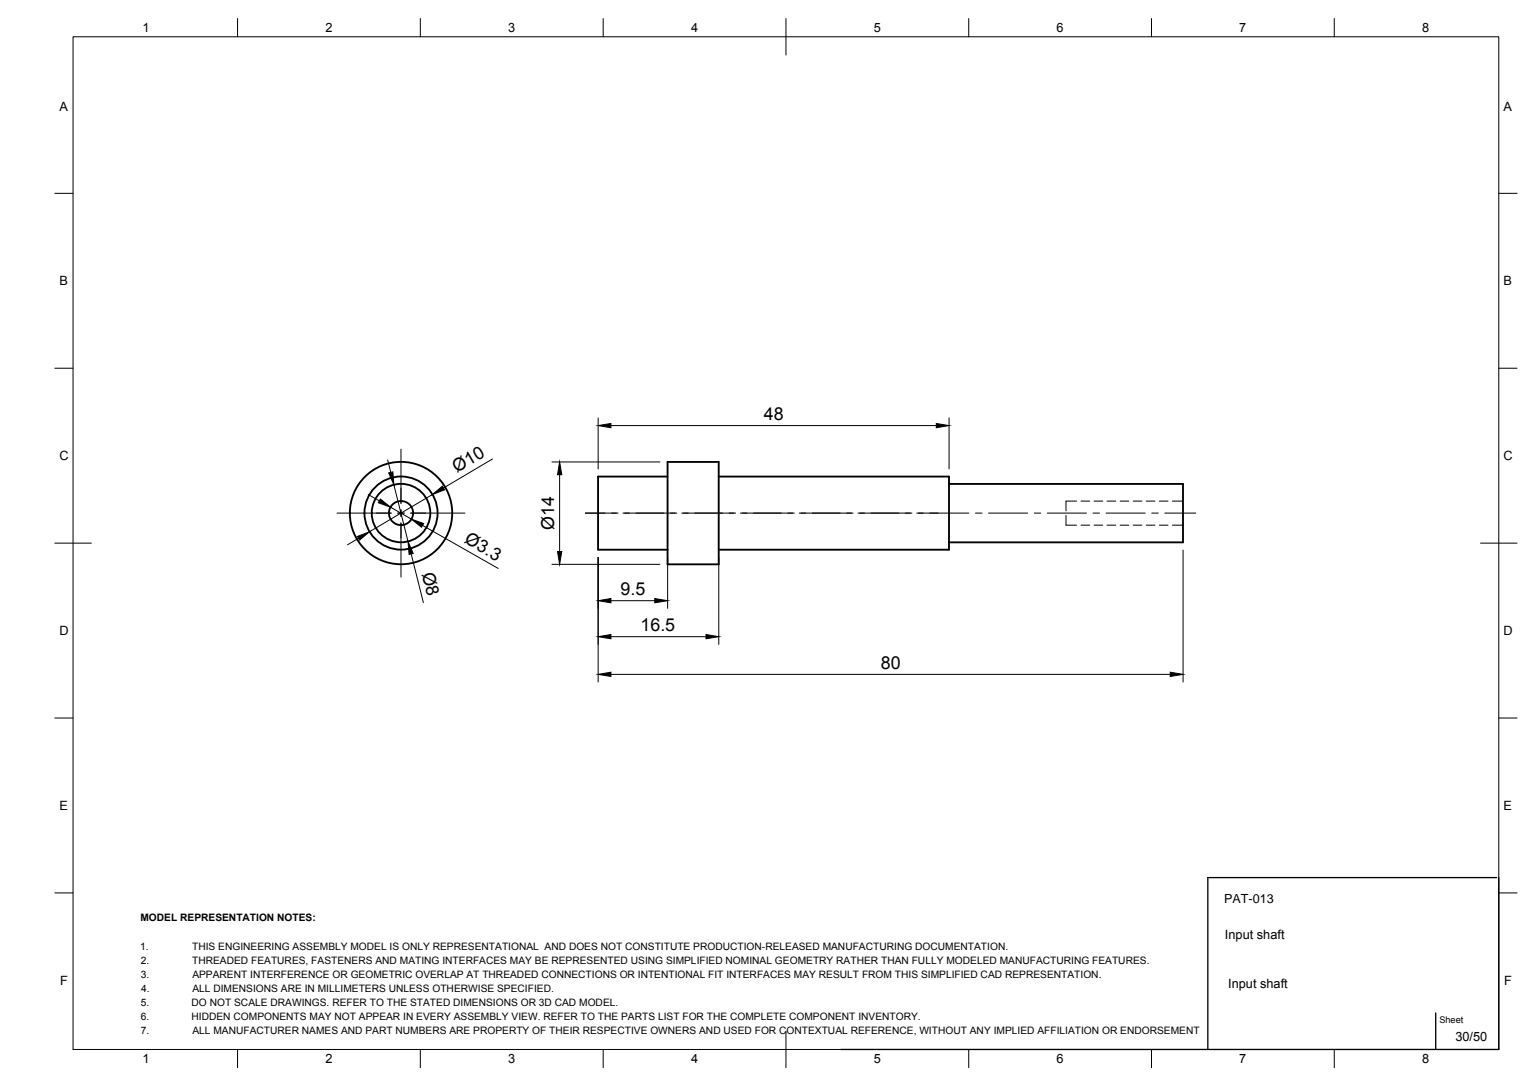
ISO-10303-21;
HEADER;
/* Generated by software containing ST-Developer
 * from STEP Tools, Inc. (www.steptools.com) 
 */

FILE_DESCRIPTION(
/* description */ ('Belt-driven linear axis on 2020 extrusion'),
/* implementation_level */ '2;1');

FILE_NAME(
/* name */ 'Input shaft.step',
/* time_stamp */ '2026-10-28T03:26:09-07:00',
/* author */ (''),
/* organization */ (''),
/* preprocessor_version */ 'ST-DEVELOPER v20.2',
/* originating_system */ 'Autodesk Translation Framework v15.17.0.0',
/* authorisation */ '');

FILE_SCHEMA (('AUTOMOTIVE_DESIGN { 1 0 10303 214 3 1 1 }'));
ENDSEC;

DATA;
#10=MECHANICAL_DESIGN_GEOMETRIC_PRESENTATION_REPRESENTATION('',(#643),#20096);
#541=SHAPE_REPRESENTATION_RELATIONSHIP('SRR','None',#20339,#587);
#587=ADVANCED_BREP_SHAPE_REPRESENTATION('',(#698),#20070);
#643=STYLED_ITEM('',(#20650),#698);
#698=MANIFOLD_SOLID_BREP('Body1',#10957);
#829=FACE_BOUND('',#2354,.T.);
#830=FACE_BOUND('',#2356,.T.);
#831=FACE_BOUND('',#2361,.T.);
#832=FACE_BOUND('',#2365,.T.);
#1110=PLANE('',#12193);
#1111=PLANE('',#12194);
#1112=PLANE('',#12197);
#1113=PLANE('',#12206);
#1114=PLANE('',#12209);
#1115=PLANE('',#12210);
#1618=FACE_OUTER_BOUND('',#2351,.T.);
#1619=FACE_OUTER_BOUND('',#2352,.T.);
#1620=FACE_OUTER_BOUND('',#2353,.T.);
#1621=FACE_OUTER_BOUND('',#2355,.T.);
#1622=FACE_OUTER_BOUND('',#2357,.T.);
#1623=FACE_OUTER_BOUND('',#2358,.T.);
#1624=FACE_OUTER_BOUND('',#2359,.T.);
#1625=FACE_OUTER_BOUND('',#2360,.T.);
#1626=FACE_OUTER_BOUND('',#2362,.T.);
#1627=FACE_OUTER_BOUND('',#2363,.T.);
#1628=FACE_OUTER_BOUND('',#2364,.T.);
#2351=EDGE_LOOP('',(#8965,#8966,#8967,#8968));
#2352=EDGE_LOOP('',(#8969));
#2353=EDGE_LOOP('',(#8970));
#2354=EDGE_LOOP('',(#8971));
#2355=EDGE_LOOP('',(#8972));
#2356=EDGE_LOOP('',(#8973));
#2357=EDGE_LOOP('',(#8974,#8975,#8976,#8977));
#2358=EDGE_LOOP('',(#8978,#8979,#8980,#8981));
#2359=EDGE_LOOP('',(#8982,#8983,#8984,#8985));
#2360=EDGE_LOOP('',(#8986));
#2361=EDGE_LOOP('',(#8987));
#2362=EDGE_LOOP('',(#8988,#8989,#8990,#8991));
#2363=EDGE_LOOP('',(#8992));
#2364=EDGE_LOOP('',(#8993));
#2365=EDGE_LOOP('',(#8994));
#3204=LINE('',#18410,#4061);
#3205=LINE('',#18424,#4062);
#3206=LINE('',#18427,#4063);
#3207=LINE('',#18433,#4064);
#3208=LINE('',#18439,#4065);
#4061=VECTOR('',#14728,0.165);
#4062=VECTOR('',#14747,0.7);
#4063=VECTOR('',#14750,0.5);
#4064=VECTOR('',#14757,0.4);
#4065=VECTOR('',#14766,0.5);
#4676=CIRCLE('',#12191,0.165);
#4677=CIRCLE('',#12192,0.165);
#4678=CIRCLE('',#12195,0.7);
#4679=CIRCLE('',#12196,0.5);
#4680=CIRCLE('',#12198,0.7);
#4681=CIRCLE('',#12199,0.5);
#4682=CIRCLE('',#12202,0.5);
#4683=CIRCLE('',#12204,0.4);
#4684=CIRCLE('',#12205,0.4);
#4685=CIRCLE('',#12208,0.5);
#5471=VERTEX_POINT('',#18407);
#5472=VERTEX_POINT('',#18409);
#5473=VERTEX_POINT('',#18414);
#5474=VERTEX_POINT('',#18416);
#5475=VERTEX_POINT('',#18419);
#5476=VERTEX_POINT('',#18421);
#5477=VERTEX_POINT('',#18426);
#5478=VERTEX_POINT('',#18430);
#5479=VERTEX_POINT('',#18432);
#5480=VERTEX_POINT('',#18437);
#6697=EDGE_CURVE('',#5471,#5471,#4676,.T.);
#6698=EDGE_CURVE('',#5471,#5472,#3204,.T.);
#6699=EDGE_CURVE('',#5472,#5472,#4677,.T.);
#6700=EDGE_CURVE('',#5473,#5473,#4678,.T.);
#6701=EDGE_CURVE('',#5474,#5474,#4679,.T.);
#6702=EDGE_CURVE('',#5475,#5475,#4680,.T.);
#6703=EDGE_CURVE('',#5476,#5476,#4681,.T.);
#6704=EDGE_CURVE('',#5473,#5475,#3205,.T.);
#6705=EDGE_CURVE('',#5476,#5477,#3206,.T.);
#6706=EDGE_CURVE('',#5477,#5477,#4682,.T.);
#6707=EDGE_CURVE('',#5478,#5478,#4683,.T.);
#6708=EDGE_CURVE('',#5478,#5479,#3207,.T.);
#6709=EDGE_CURVE('',#5479,#5479,#4684,.T.);
#6710=EDGE_CURVE('',#5480,#5480,#4685,.T.);
#6711=EDGE_CURVE('',#5480,#5474,#3208,.T.);
#8965=ORIENTED_EDGE('',*,*,#6697,.F.);
#8966=ORIENTED_EDGE('',*,*,#6698,.T.);
#8967=ORIENTED_EDGE('',*,*,#6699,.T.);
#8968=ORIENTED_EDGE('',*,*,#6698,.F.);
#8969=ORIENTED_EDGE('',*,*,#6699,.F.);
#8970=ORIENTED_EDGE('',*,*,#6700,.T.);
#8971=ORIENTED_EDGE('',*,*,#6701,.F.);
#8972=ORIENTED_EDGE('',*,*,#6702,.F.);
#8973=ORIENTED_EDGE('',*,*,#6703,.F.);
#8974=ORIENTED_EDGE('',*,*,#6700,.F.);
#8975=ORIENTED_EDGE('',*,*,#6704,.T.);
#8976=ORIENTED_EDGE('',*,*,#6702,.T.);
#8977=ORIENTED_EDGE('',*,*,#6704,.F.);
#8978=ORIENTED_EDGE('',*,*,#6703,.T.);
#8979=ORIENTED_EDGE('',*,*,#6705,.T.);
#8980=ORIENTED_EDGE('',*,*,#6706,.T.);
#8981=ORIENTED_EDGE('',*,*,#6705,.F.);
#8982=ORIENTED_EDGE('',*,*,#6707,.F.);
#8983=ORIENTED_EDGE('',*,*,#6708,.T.);
#8984=ORIENTED_EDGE('',*,*,#6709,.T.);
#8985=ORIENTED_EDGE('',*,*,#6708,.F.);
#8986=ORIENTED_EDGE('',*,*,#6709,.F.);
#8987=ORIENTED_EDGE('',*,*,#6697,.T.);
#8988=ORIENTED_EDGE('',*,*,#6710,.F.);
#8989=ORIENTED_EDGE('',*,*,#6711,.T.);
#8990=ORIENTED_EDGE('',*,*,#6701,.T.);
#8991=ORIENTED_EDGE('',*,*,#6711,.F.);
#8992=ORIENTED_EDGE('',*,*,#6710,.T.);
#8993=ORIENTED_EDGE('',*,*,#6706,.F.);
#8994=ORIENTED_EDGE('',*,*,#6707,.T.);
#10199=CYLINDRICAL_SURFACE('',#12190,0.165);
#10200=CYLINDRICAL_SURFACE('',#12200,0.7);
#10201=CYLINDRICAL_SURFACE('',#12201,0.5);
#10202=CYLINDRICAL_SURFACE('',#12203,0.4);
#10203=CYLINDRICAL_SURFACE('',#12207,0.5);
#10669=ADVANCED_FACE('',(#1618),#10199,.F.);
#10670=ADVANCED_FACE('',(#1619),#1110,.F.);
#10671=ADVANCED_FACE('',(#1620,#829),#1111,.T.);
#10672=ADVANCED_FACE('',(#1621,#830),#1112,.F.);
#10673=ADVANCED_FACE('',(#1622),#10200,.T.);
#10674=ADVANCED_FACE('',(#1623),#10201,.T.);
#10675=ADVANCED_FACE('',(#1624),#10202,.T.);
#10676=ADVANCED_FACE('',(#1625,#831),#1113,.F.);
#10677=ADVANCED_FACE('',(#1626),#10203,.T.);
#10678=ADVANCED_FACE('',(#1627),#1114,.T.);
#10679=ADVANCED_FACE('',(#1628,#832),#1115,.F.);
#10957=CLOSED_SHELL('',(#10669,#10670,#10671,#10672,#10673,#10674,#10675,
#10676,#10677,#10678,#10679));
#12189=AXIS2_PLACEMENT_3D('',#18405,#14722,#14723);
#12190=AXIS2_PLACEMENT_3D('',#18406,#14724,#14725);
#12191=AXIS2_PLACEMENT_3D('',#18408,#14726,#14727);
#12192=AXIS2_PLACEMENT_3D('',#18411,#14729,#14730);
#12193=AXIS2_PLACEMENT_3D('',#18412,#14731,#14732);
#12194=AXIS2_PLACEMENT_3D('',#18413,#14733,#14734);
#12195=AXIS2_PLACEMENT_3D('',#18415,#14735,#14736);
#12196=AXIS2_PLACEMENT_3D('',#18417,#14737,#14738);
#12197=AXIS2_PLACEMENT_3D('',#18418,#14739,#14740);
#12198=AXIS2_PLACEMENT_3D('',#18420,#14741,#14742);
#12199=AXIS2_PLACEMENT_3D('',#18422,#14743,#14744);
#12200=AXIS2_PLACEMENT_3D('',#18423,#14745,#14746);
#12201=AXIS2_PLACEMENT_3D('',#18425,#14748,#14749);
#12202=AXIS2_PLACEMENT_3D('',#18428,#14751,#14752);
#12203=AXIS2_PLACEMENT_3D('',#18429,#14753,#14754);
#12204=AXIS2_PLACEMENT_3D('',#18431,#14755,#14756);
#12205=AXIS2_PLACEMENT_3D('',#18434,#14758,#14759);
#12206=AXIS2_PLACEMENT_3D('',#18435,#14760,#14761);
#12207=AXIS2_PLACEMENT_3D('',#18436,#14762,#14763);
#12208=AXIS2_PLACEMENT_3D('',#18438,#14764,#14765);
#12209=AXIS2_PLACEMENT_3D('',#18440,#14767,#14768);
#12210=AXIS2_PLACEMENT_3D('',#18441,#14769,#14770);
#14722=DIRECTION('axis',(0.,0.,1.));
#14723=DIRECTION('refdir',(1.,0.,0.));
#14724=DIRECTION('center_axis',(0.,1.,0.));
#14725=DIRECTION('ref_axis',(1.,0.,0.));
#14726=DIRECTION('center_axis',(0.,1.,0.));
#14727=DIRECTION('ref_axis',(1.,0.,0.));
#14728=DIRECTION('',(0.,1.,0.));
#14729=DIRECTION('center_axis',(0.,1.,0.));
#14730=DIRECTION('ref_axis',(1.,0.,0.));
#14731=DIRECTION('center_axis',(0.,1.,0.));
#14732=DIRECTION('ref_axis',(1.,0.,0.));
#14733=DIRECTION('center_axis',(0.,1.,0.));
#14734=DIRECTION('ref_axis',(1.,0.,0.));
#14735=DIRECTION('center_axis',(0.,1.,0.));
#14736=DIRECTION('ref_axis',(1.,0.,0.));
#14737=DIRECTION('center_axis',(0.,1.,0.));
#14738=DIRECTION('ref_axis',(1.,0.,0.));
#14739=DIRECTION('center_axis',(0.,1.,0.));
#14740=DIRECTION('ref_axis',(1.,0.,0.));
#14741=DIRECTION('center_axis',(0.,1.,0.));
#14742=DIRECTION('ref_axis',(1.,0.,0.));
#14743=DIRECTION('center_axis',(0.,-1.,0.));
#14744=DIRECTION('ref_axis',(1.,0.,0.));
#14745=DIRECTION('center_axis',(0.,1.,0.));
#14746=DIRECTION('ref_axis',(1.,0.,0.));
#14747=DIRECTION('',(0.,-1.,0.));
#14748=DIRECTION('center_axis',(0.,1.,0.));
#14749=DIRECTION('ref_axis',(1.,0.,0.));
#14750=DIRECTION('',(0.,-1.,0.));
#14751=DIRECTION('center_axis',(0.,1.,0.));
#14752=DIRECTION('ref_axis',(1.,0.,0.));
#14753=DIRECTION('center_axis',(0.,1.,0.));
#14754=DIRECTION('ref_axis',(1.,0.,0.));
#14755=DIRECTION('center_axis',(0.,1.,0.));
#14756=DIRECTION('ref_axis',(1.,0.,0.));
#14757=DIRECTION('',(0.,-1.,0.));
#14758=DIRECTION('center_axis',(0.,1.,0.));
#14759=DIRECTION('ref_axis',(1.,0.,0.));
#14760=DIRECTION('center_axis',(0.,1.,0.));
#14761=DIRECTION('ref_axis',(1.,0.,0.));
#14762=DIRECTION('center_axis',(0.,1.,0.));
#14763=DIRECTION('ref_axis',(1.,0.,0.));
#14764=DIRECTION('center_axis',(0.,1.,0.));
#14765=DIRECTION('ref_axis',(1.,0.,0.));
#14766=DIRECTION('',(0.,-1.,0.));
#14767=DIRECTION('center_axis',(0.,1.,0.));
#14768=DIRECTION('ref_axis',(1.,0.,0.));
#14769=DIRECTION('center_axis',(0.,1.,0.));
#14770=DIRECTION('ref_axis',(1.,0.,0.));
#18405=CARTESIAN_POINT('',(0.,0.,0.));
#18406=CARTESIAN_POINT('Origin',(0.,-5.1,7.));
#18407=CARTESIAN_POINT('',(-0.165,-5.,7.));
#18408=CARTESIAN_POINT('Origin',(0.,-5.,7.));
#18409=CARTESIAN_POINT('',(-0.165,-3.4,7.));
#18410=CARTESIAN_POINT('',(-0.165,-5.1,7.));
#18411=CARTESIAN_POINT('Origin',(0.,-3.4,7.));
#18412=CARTESIAN_POINT('Origin',(0.,-3.4,7.));
#18413=CARTESIAN_POINT('Origin',(0.,2.05,7.));
#18414=CARTESIAN_POINT('',(-0.7,2.05,7.));
#18415=CARTESIAN_POINT('Origin',(0.,2.05,7.));
#18416=CARTESIAN_POINT('',(-0.5,2.05,7.));
#18417=CARTESIAN_POINT('Origin',(0.,2.05,7.));
#18418=CARTESIAN_POINT('Origin',(0.,1.35,7.));
#18419=CARTESIAN_POINT('',(-0.7,1.35,7.));
#18420=CARTESIAN_POINT('Origin',(0.,1.35,7.));
#18421=CARTESIAN_POINT('',(-0.5,1.35,7.));
#18422=CARTESIAN_POINT('Origin',(0.,1.35,7.));
#18423=CARTESIAN_POINT('Origin',(0.,1.35,7.));
#18424=CARTESIAN_POINT('',(-0.7,1.35,7.));
#18425=CARTESIAN_POINT('Origin',(0.,-1.8,7.));
#18426=CARTESIAN_POINT('',(-0.5,-1.8,7.));
#18427=CARTESIAN_POINT('',(-0.5,-1.8,7.));
#18428=CARTESIAN_POINT('Origin',(0.,-1.8,7.));
#18429=CARTESIAN_POINT('Origin',(0.,-5.,7.));
#18430=CARTESIAN_POINT('',(-0.4,-1.8,7.));
#18431=CARTESIAN_POINT('Origin',(0.,-1.8,7.));
#18432=CARTESIAN_POINT('',(-0.4,-5.,7.));
#18433=CARTESIAN_POINT('',(-0.4,-5.,7.));
#18434=CARTESIAN_POINT('Origin',(0.,-5.,7.));
#18435=CARTESIAN_POINT('Origin',(0.,-5.,7.));
#18436=CARTESIAN_POINT('Origin',(0.,-1.8,7.));
#18437=CARTESIAN_POINT('',(-0.5,3.,7.));
#18438=CARTESIAN_POINT('Origin',(0.,3.,7.));
#18439=CARTESIAN_POINT('',(-0.5,-1.8,7.));
#18440=CARTESIAN_POINT('Origin',(0.,3.,7.));
#18441=CARTESIAN_POINT('Origin',(0.,-1.8,7.));
#20016=UNCERTAINTY_MEASURE_WITH_UNIT(LENGTH_MEASURE(0.001),#20097,
'DISTANCE_ACCURACY_VALUE',
'Maximum model space distance between geometric entities at asserted c
onnectivities');
#20042=UNCERTAINTY_MEASURE_WITH_UNIT(LENGTH_MEASURE(0.001),#20097,
'DISTANCE_ACCURACY_VALUE',
'Maximum model space distance between geometric entities at asserted c
onnectivities');
#20070=(
GEOMETRIC_REPRESENTATION_CONTEXT(3)
GLOBAL_UNCERTAINTY_ASSIGNED_CONTEXT((#20016))
GLOBAL_UNIT_ASSIGNED_CONTEXT((#20097,#20099,#20100))
REPRESENTATION_CONTEXT('','3D')
);
#20096=(
GEOMETRIC_REPRESENTATION_CONTEXT(3)
GLOBAL_UNCERTAINTY_ASSIGNED_CONTEXT((#20042))
GLOBAL_UNIT_ASSIGNED_CONTEXT((#20097,#20099,#20100))
REPRESENTATION_CONTEXT('','3D')
);
#20097=(
LENGTH_UNIT()
NAMED_UNIT(*)
SI_UNIT(.CENTI.,.METRE.)
);
#20099=(
NAMED_UNIT(*)
PLANE_ANGLE_UNIT()
SI_UNIT($,.RADIAN.)
);
#20100=(
NAMED_UNIT(*)
SI_UNIT($,.STERADIAN.)
SOLID_ANGLE_UNIT()
);
#20128=SHAPE_DEFINITION_REPRESENTATION(#20186,#20339);
#20186=PRODUCT_DEFINITION_SHAPE('',$,#20393);
#20339=SHAPE_REPRESENTATION('',(#12189),#20070);
#20365=PRODUCT_DEFINITION_CONTEXT('part definition',#20526,'design');
#20393=PRODUCT_DEFINITION('Input shaft','Input shaft',#20446,#20365);
#20446=PRODUCT_DEFINITION_FORMATION('',$,#20555);
#20526=APPLICATION_CONTEXT(
'Core Data for Automotive Mechanical Design Process');
#20527=PRODUCT_CONTEXT('part definition',#20526,'mechanical');
#20555=PRODUCT('Input shaft','Input shaft','Input shaft',(#20527));
#20644=COLOUR_RGB('Grey',0.48,0.52,0.57);
#20645=FILL_AREA_STYLE_COLOUR('',#20644);
#20646=FILL_AREA_STYLE('',(#20645));
#20647=SURFACE_STYLE_FILL_AREA(#20646);
#20648=SURFACE_SIDE_STYLE('',(#20647));
#20649=SURFACE_STYLE_USAGE(.BOTH.,#20648);
#20650=PRESENTATION_STYLE_ASSIGNMENT((#20649));
ENDSEC;
END-ISO-10303-21;
